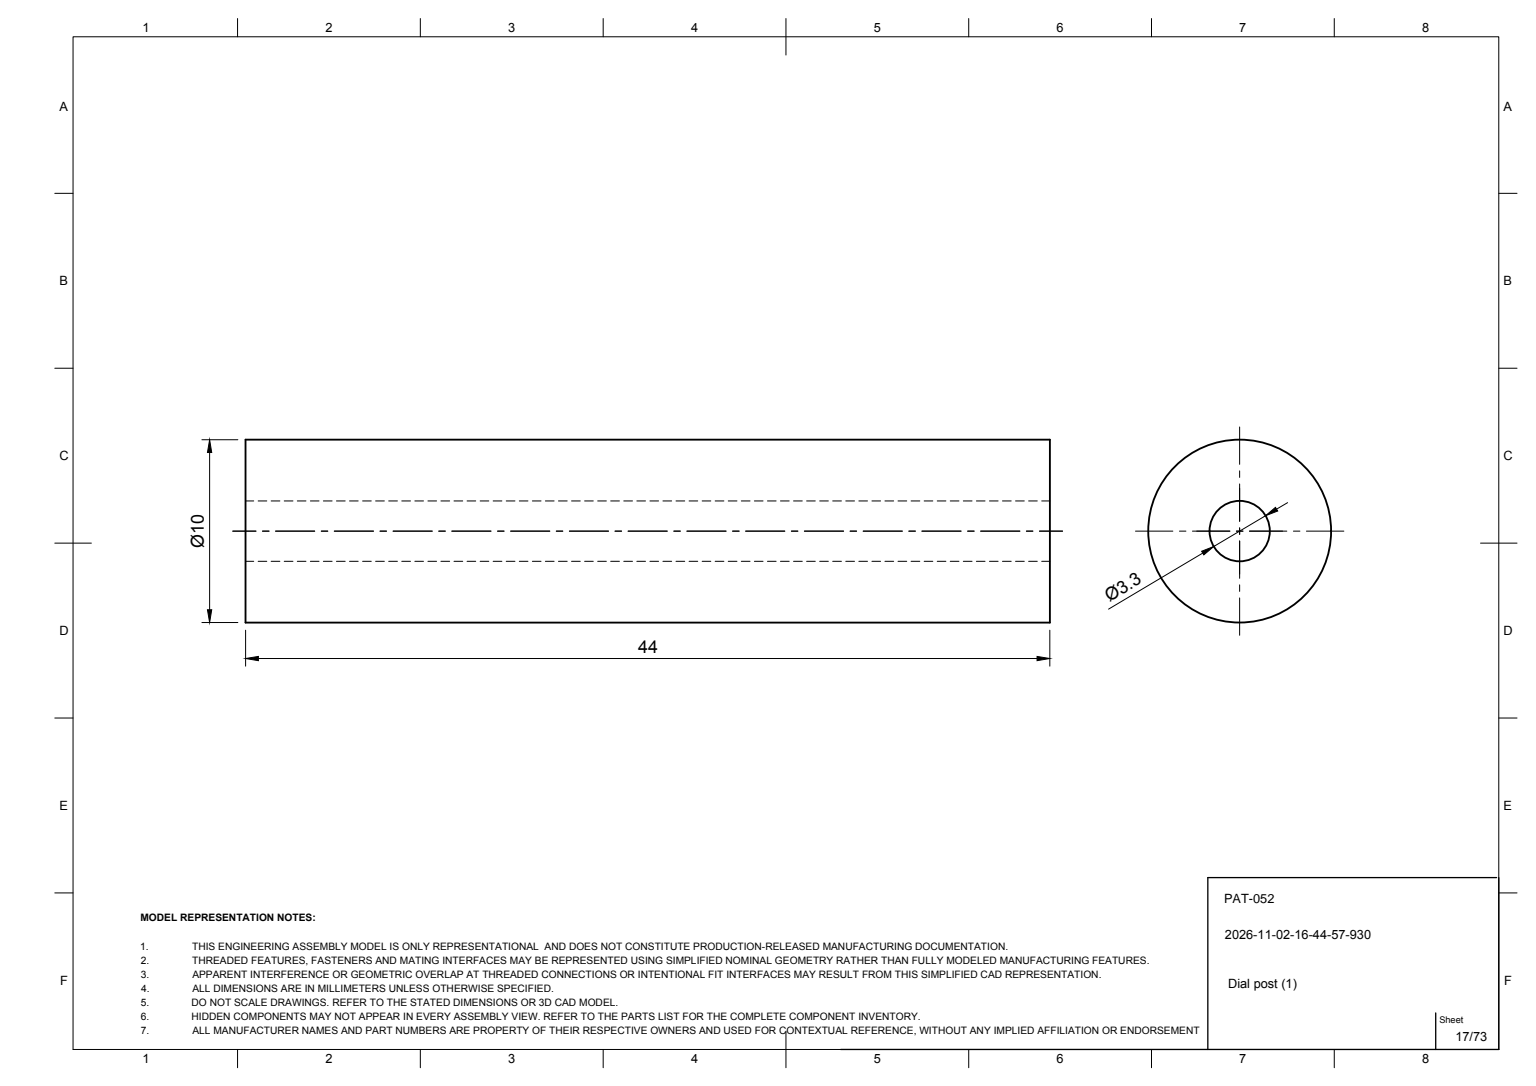
ISO-10303-21;
HEADER;
/* Generated by software containing ST-Developer
 * from STEP Tools, Inc. (www.steptools.com) 
 */

FILE_DESCRIPTION(
/* description */ ('Hand-crank gear train demonstrator'),
/* implementation_level */ '2;1');

FILE_NAME(
/* name */ 'Dial post (1).step',
/* time_stamp */ '2026-10-28T03:22:13-07:00',
/* author */ (''),
/* organization */ (''),
/* preprocessor_version */ 'ST-DEVELOPER v20.2',
/* originating_system */ 'Autodesk Translation Framework v15.17.0.0',
/* authorisation */ '');

FILE_SCHEMA (('AUTOMOTIVE_DESIGN { 1 0 10303 214 3 1 1 }'));
ENDSEC;

DATA;
#10=MECHANICAL_DESIGN_GEOMETRIC_PRESENTATION_REPRESENTATION('',(#1228),#62758);
#1085=SHAPE_REPRESENTATION_RELATIONSHIP('SRR','None',#63059,#1149);
#1149=ADVANCED_BREP_SHAPE_REPRESENTATION('',(#1305),#62713);
#1228=STYLED_ITEM('',(#63455),#1305);
#1305=MANIFOLD_SOLID_BREP('Body1',#16410);
#1538=FACE_BOUND('',#3648,.T.);
#1539=FACE_BOUND('',#3650,.T.);
#1857=PLANE('',#17928);
#1858=PLANE('',#17929);
#2513=FACE_OUTER_BOUND('',#3645,.T.);
#2514=FACE_OUTER_BOUND('',#3646,.T.);
#2515=FACE_OUTER_BOUND('',#3647,.T.);
#2516=FACE_OUTER_BOUND('',#3649,.T.);
#3645=EDGE_LOOP('',(#12583,#12584,#12585,#12586));
#3646=EDGE_LOOP('',(#12587,#12588,#12589,#12590));
#3647=EDGE_LOOP('',(#12591));
#3648=EDGE_LOOP('',(#12592));
#3649=EDGE_LOOP('',(#12593));
#3650=EDGE_LOOP('',(#12594));
#4793=LINE('',#25846,#5925);
#4794=LINE('',#25852,#5926);
#5925=VECTOR('',#20870,0.164999999999999);
#5926=VECTOR('',#20877,0.5);
#6885=CIRCLE('',#17923,0.164999999999999);
#6886=CIRCLE('',#17924,0.164999999999999);
#6887=CIRCLE('',#17926,0.5);
#6888=CIRCLE('',#17927,0.5);
#7810=VERTEX_POINT('',#25843);
#7811=VERTEX_POINT('',#25845);
#7812=VERTEX_POINT('',#25849);
#7813=VERTEX_POINT('',#25851);
#9543=EDGE_CURVE('',#7810,#7810,#6885,.T.);
#9544=EDGE_CURVE('',#7810,#7811,#4793,.T.);
#9545=EDGE_CURVE('',#7811,#7811,#6886,.T.);
#9546=EDGE_CURVE('',#7812,#7812,#6887,.T.);
#9547=EDGE_CURVE('',#7812,#7813,#4794,.T.);
#9548=EDGE_CURVE('',#7813,#7813,#6888,.T.);
#12583=ORIENTED_EDGE('',*,*,#9543,.F.);
#12584=ORIENTED_EDGE('',*,*,#9544,.T.);
#12585=ORIENTED_EDGE('',*,*,#9545,.F.);
#12586=ORIENTED_EDGE('',*,*,#9544,.F.);
#12587=ORIENTED_EDGE('',*,*,#9546,.F.);
#12588=ORIENTED_EDGE('',*,*,#9547,.T.);
#12589=ORIENTED_EDGE('',*,*,#9548,.T.);
#12590=ORIENTED_EDGE('',*,*,#9547,.F.);
#12591=ORIENTED_EDGE('',*,*,#9546,.T.);
#12592=ORIENTED_EDGE('',*,*,#9545,.T.);
#12593=ORIENTED_EDGE('',*,*,#9548,.F.);
#12594=ORIENTED_EDGE('',*,*,#9543,.T.);
#15285=CYLINDRICAL_SURFACE('',#17922,0.164999999999999);
#15286=CYLINDRICAL_SURFACE('',#17925,0.5);
#15823=ADVANCED_FACE('',(#2513),#15285,.F.);
#15824=ADVANCED_FACE('',(#2514),#15286,.T.);
#15825=ADVANCED_FACE('',(#2515,#1538),#1857,.T.);
#15826=ADVANCED_FACE('',(#2516,#1539),#1858,.F.);
#16410=CLOSED_SHELL('',(#15823,#15824,#15825,#15826));
#17921=AXIS2_PLACEMENT_3D('',#25841,#20864,#20865);
#17922=AXIS2_PLACEMENT_3D('',#25842,#20866,#20867);
#17923=AXIS2_PLACEMENT_3D('',#25844,#20868,#20869);
#17924=AXIS2_PLACEMENT_3D('',#25847,#20871,#20872);
#17925=AXIS2_PLACEMENT_3D('',#25848,#20873,#20874);
#17926=AXIS2_PLACEMENT_3D('',#25850,#20875,#20876);
#17927=AXIS2_PLACEMENT_3D('',#25853,#20878,#20879);
#17928=AXIS2_PLACEMENT_3D('',#25854,#20880,#20881);
#17929=AXIS2_PLACEMENT_3D('',#25855,#20882,#20883);
#20864=DIRECTION('axis',(0.,0.,1.));
#20865=DIRECTION('refdir',(1.,0.,0.));
#20866=DIRECTION('center_axis',(0.,1.,0.));
#20867=DIRECTION('ref_axis',(1.,0.,0.));
#20868=DIRECTION('center_axis',(0.,1.,0.));
#20869=DIRECTION('ref_axis',(1.,0.,0.));
#20870=DIRECTION('',(0.,1.,0.));
#20871=DIRECTION('center_axis',(0.,-1.,0.));
#20872=DIRECTION('ref_axis',(1.,0.,0.));
#20873=DIRECTION('center_axis',(0.,1.,0.));
#20874=DIRECTION('ref_axis',(1.,0.,0.));
#20875=DIRECTION('center_axis',(0.,1.,0.));
#20876=DIRECTION('ref_axis',(1.,0.,0.));
#20877=DIRECTION('',(0.,-1.,0.));
#20878=DIRECTION('center_axis',(0.,1.,0.));
#20879=DIRECTION('ref_axis',(1.,0.,0.));
#20880=DIRECTION('center_axis',(0.,1.,0.));
#20881=DIRECTION('ref_axis',(1.,0.,0.));
#20882=DIRECTION('center_axis',(0.,1.,0.));
#20883=DIRECTION('ref_axis',(1.,0.,0.));
#25841=CARTESIAN_POINT('',(0.,0.,0.));
#25842=CARTESIAN_POINT('Origin',(23.,-0.7,14.));
#25843=CARTESIAN_POINT('',(22.835,-0.6,14.));
#25844=CARTESIAN_POINT('Origin',(23.,-0.6,14.));
#25845=CARTESIAN_POINT('',(22.835,3.8,14.));
#25846=CARTESIAN_POINT('',(22.835,-0.7,14.));
#25847=CARTESIAN_POINT('Origin',(23.,3.8,14.));
#25848=CARTESIAN_POINT('Origin',(23.,-0.6,14.));
#25849=CARTESIAN_POINT('',(22.5,3.8,14.));
#25850=CARTESIAN_POINT('Origin',(23.,3.8,14.));
#25851=CARTESIAN_POINT('',(22.5,-0.6,14.));
#25852=CARTESIAN_POINT('',(22.5,-0.6,14.));
#25853=CARTESIAN_POINT('Origin',(23.,-0.6,14.));
#25854=CARTESIAN_POINT('Origin',(23.,3.8,14.));
#25855=CARTESIAN_POINT('Origin',(23.,-0.6,14.));
#62639=UNCERTAINTY_MEASURE_WITH_UNIT(LENGTH_MEASURE(0.001),#62759,
'DISTANCE_ACCURACY_VALUE',
'Maximum model space distance between geometric entities at asserted c
onnectivities');
#62684=UNCERTAINTY_MEASURE_WITH_UNIT(LENGTH_MEASURE(0.001),#62759,
'DISTANCE_ACCURACY_VALUE',
'Maximum model space distance between geometric entities at asserted c
onnectivities');
#62713=(
GEOMETRIC_REPRESENTATION_CONTEXT(3)
GLOBAL_UNCERTAINTY_ASSIGNED_CONTEXT((#62639))
GLOBAL_UNIT_ASSIGNED_CONTEXT((#62759,#62761,#62762))
REPRESENTATION_CONTEXT('','3D')
);
#62758=(
GEOMETRIC_REPRESENTATION_CONTEXT(3)
GLOBAL_UNCERTAINTY_ASSIGNED_CONTEXT((#62684))
GLOBAL_UNIT_ASSIGNED_CONTEXT((#62759,#62761,#62762))
REPRESENTATION_CONTEXT('','3D')
);
#62759=(
LENGTH_UNIT()
NAMED_UNIT(*)
SI_UNIT(.CENTI.,.METRE.)
);
#62761=(
NAMED_UNIT(*)
PLANE_ANGLE_UNIT()
SI_UNIT($,.RADIAN.)
);
#62762=(
NAMED_UNIT(*)
SI_UNIT($,.STERADIAN.)
SOLID_ANGLE_UNIT()
);
#62791=SHAPE_DEFINITION_REPRESENTATION(#62874,#63059);
#62874=PRODUCT_DEFINITION_SHAPE('',$,#63133);
#63059=SHAPE_REPRESENTATION('',(#17921),#62713);
#63104=PRODUCT_DEFINITION_CONTEXT('part definition',#63325,'design');
#63133=PRODUCT_DEFINITION('Dial post (1)','Dial post (1)',#63206,#63104);
#63206=PRODUCT_DEFINITION_FORMATION('',$,#63355);
#63325=APPLICATION_CONTEXT(
'Core Data for Automotive Mechanical Design Process');
#63326=PRODUCT_CONTEXT('part definition',#63325,'mechanical');
#63355=PRODUCT('Dial post (1)','Dial post (1)','Dial post (1)',(#63326));
#63449=COLOUR_RGB('Sky Blue',0.24,0.69,0.87);
#63450=FILL_AREA_STYLE_COLOUR('',#63449);
#63451=FILL_AREA_STYLE('',(#63450));
#63452=SURFACE_STYLE_FILL_AREA(#63451);
#63453=SURFACE_SIDE_STYLE('',(#63452));
#63454=SURFACE_STYLE_USAGE(.BOTH.,#63453);
#63455=PRESENTATION_STYLE_ASSIGNMENT((#63454));
ENDSEC;
END-ISO-10303-21;
